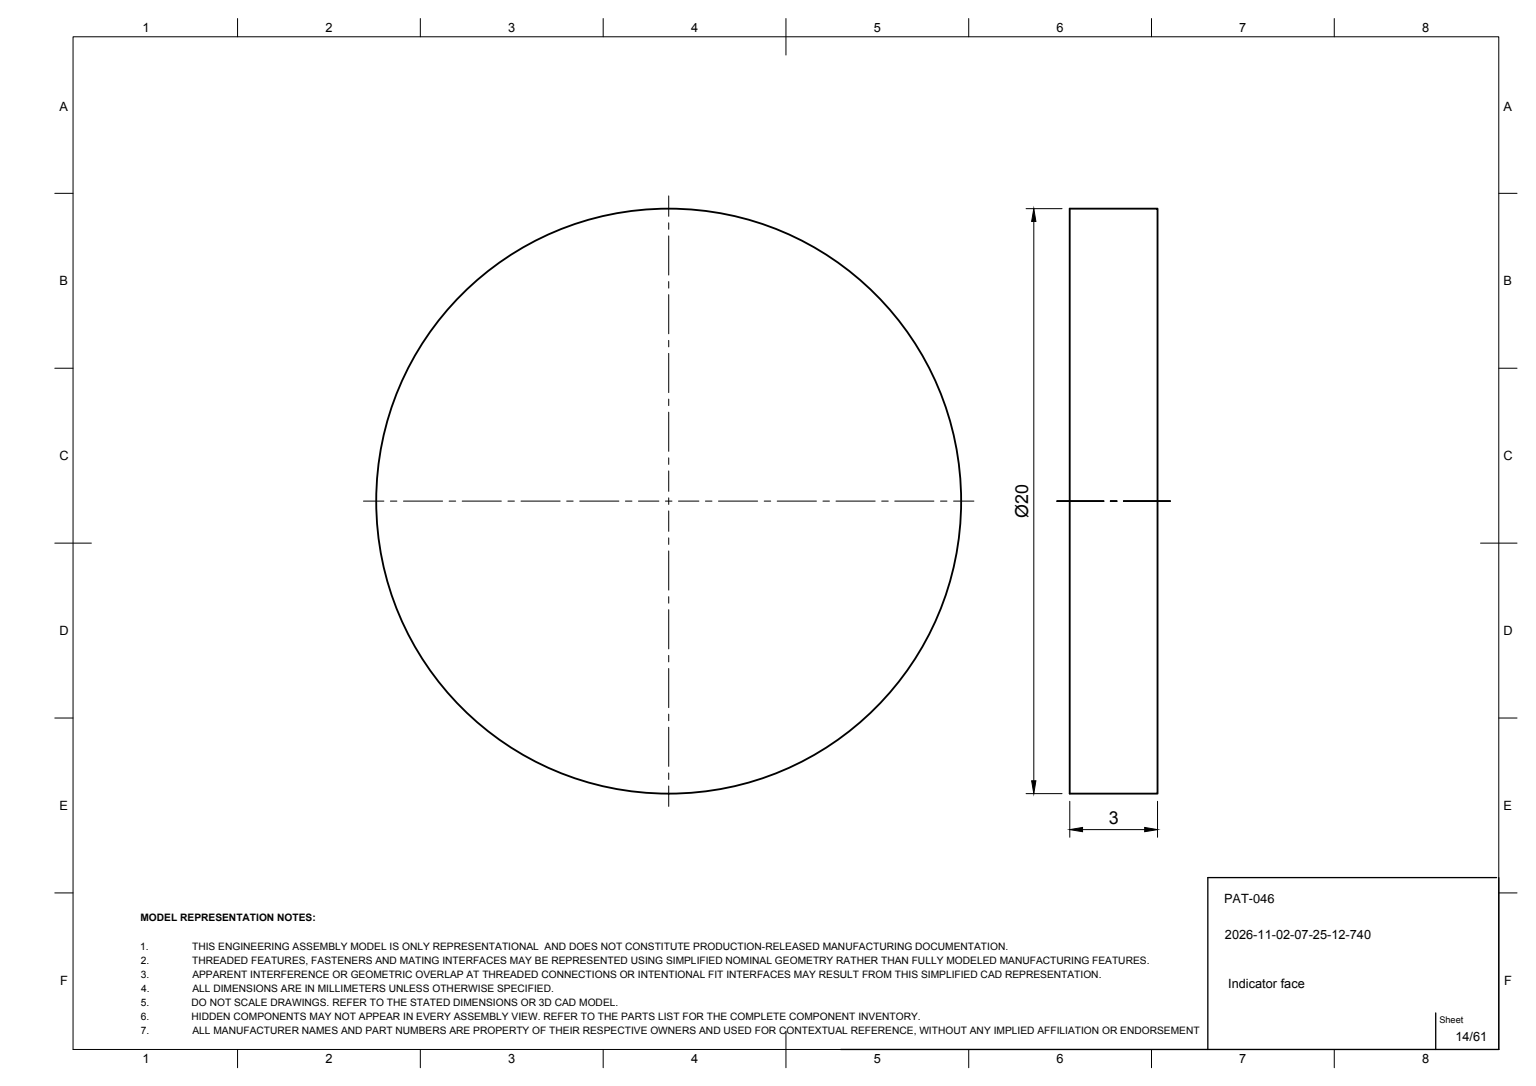
ISO-10303-21;
HEADER;
/* Generated by software containing ST-Developer
 * from STEP Tools, Inc. (www.steptools.com) 
 */

FILE_DESCRIPTION(
/* description */ ('Gear mesh backlash fixture'),
/* implementation_level */ '2;1');

FILE_NAME(
/* name */ 'Indicator face.step',
/* time_stamp */ '2026-10-28T03:26:00-07:00',
/* author */ (''),
/* organization */ (''),
/* preprocessor_version */ 'ST-DEVELOPER v20.2',
/* originating_system */ 'Autodesk Translation Framework v15.17.0.0',
/* authorisation */ '');

FILE_SCHEMA (('AUTOMOTIVE_DESIGN { 1 0 10303 214 3 1 1 }'));
ENDSEC;

DATA;
#10=MECHANICAL_DESIGN_GEOMETRIC_PRESENTATION_REPRESENTATION('',(#1025),#57900);
#925=SHAPE_REPRESENTATION_RELATIONSHIP('SRR','None',#58120,#975);
#975=ADVANCED_BREP_SHAPE_REPRESENTATION('',(#1090),#57853);
#1025=STYLED_ITEM('',(#58458),#1090);
#1090=MANIFOLD_SOLID_BREP('Body1',#13585);
#1391=PLANE('',#14445);
#1392=PLANE('',#14446);
#1808=FACE_OUTER_BOUND('',#2635,.T.);
#1809=FACE_OUTER_BOUND('',#2636,.T.);
#1810=FACE_OUTER_BOUND('',#2637,.T.);
#2635=EDGE_LOOP('',(#9415,#9416,#9417,#9418));
#2636=EDGE_LOOP('',(#9419));
#2637=EDGE_LOOP('',(#9420));
#3551=LINE('',#19900,#4440);
#4440=VECTOR('',#16216,1.);
#5310=CIRCLE('',#14443,1.);
#5311=CIRCLE('',#14444,1.);
#5955=VERTEX_POINT('',#19897);
#5956=VERTEX_POINT('',#19899);
#7294=EDGE_CURVE('',#5955,#5955,#5310,.T.);
#7295=EDGE_CURVE('',#5955,#5956,#3551,.T.);
#7296=EDGE_CURVE('',#5956,#5956,#5311,.T.);
#9415=ORIENTED_EDGE('',*,*,#7294,.F.);
#9416=ORIENTED_EDGE('',*,*,#7295,.T.);
#9417=ORIENTED_EDGE('',*,*,#7296,.T.);
#9418=ORIENTED_EDGE('',*,*,#7295,.F.);
#9419=ORIENTED_EDGE('',*,*,#7294,.T.);
#9420=ORIENTED_EDGE('',*,*,#7296,.F.);
#12638=CYLINDRICAL_SURFACE('',#14442,1.);
#12925=ADVANCED_FACE('',(#1808),#12638,.T.);
#12926=ADVANCED_FACE('',(#1809),#1391,.T.);
#12927=ADVANCED_FACE('',(#1810),#1392,.F.);
#13585=CLOSED_SHELL('',(#12925,#12926,#12927));
#14441=AXIS2_PLACEMENT_3D('',#19895,#16210,#16211);
#14442=AXIS2_PLACEMENT_3D('',#19896,#16212,#16213);
#14443=AXIS2_PLACEMENT_3D('',#19898,#16214,#16215);
#14444=AXIS2_PLACEMENT_3D('',#19901,#16217,#16218);
#14445=AXIS2_PLACEMENT_3D('',#19902,#16219,#16220);
#14446=AXIS2_PLACEMENT_3D('',#19903,#16221,#16222);
#16210=DIRECTION('axis',(0.,0.,1.));
#16211=DIRECTION('refdir',(1.,0.,0.));
#16212=DIRECTION('center_axis',(0.,1.,0.));
#16213=DIRECTION('ref_axis',(1.,0.,0.));
#16214=DIRECTION('center_axis',(0.,1.,0.));
#16215=DIRECTION('ref_axis',(1.,0.,0.));
#16216=DIRECTION('',(0.,-1.,0.));
#16217=DIRECTION('center_axis',(0.,1.,0.));
#16218=DIRECTION('ref_axis',(1.,0.,0.));
#16219=DIRECTION('center_axis',(0.,1.,0.));
#16220=DIRECTION('ref_axis',(1.,0.,0.));
#16221=DIRECTION('center_axis',(0.,1.,0.));
#16222=DIRECTION('ref_axis',(1.,0.,0.));
#19895=CARTESIAN_POINT('',(0.,0.,0.));
#19896=CARTESIAN_POINT('Origin',(6.,10.,12.));
#19897=CARTESIAN_POINT('',(5.,10.3,12.));
#19898=CARTESIAN_POINT('Origin',(6.,10.3,12.));
#19899=CARTESIAN_POINT('',(5.,10.,12.));
#19900=CARTESIAN_POINT('',(5.,10.,12.));
#19901=CARTESIAN_POINT('Origin',(6.,10.,12.));
#19902=CARTESIAN_POINT('Origin',(6.,10.3,12.));
#19903=CARTESIAN_POINT('Origin',(6.,10.,12.));
#57794=UNCERTAINTY_MEASURE_WITH_UNIT(LENGTH_MEASURE(0.001),#57901,
'DISTANCE_ACCURACY_VALUE',
'Maximum model space distance between geometric entities at asserted c
onnectivities');
#57841=UNCERTAINTY_MEASURE_WITH_UNIT(LENGTH_MEASURE(0.001),#57901,
'DISTANCE_ACCURACY_VALUE',
'Maximum model space distance between geometric entities at asserted c
onnectivities');
#57853=(
GEOMETRIC_REPRESENTATION_CONTEXT(3)
GLOBAL_UNCERTAINTY_ASSIGNED_CONTEXT((#57794))
GLOBAL_UNIT_ASSIGNED_CONTEXT((#57901,#57903,#57904))
REPRESENTATION_CONTEXT('','3D')
);
#57900=(
GEOMETRIC_REPRESENTATION_CONTEXT(3)
GLOBAL_UNCERTAINTY_ASSIGNED_CONTEXT((#57841))
GLOBAL_UNIT_ASSIGNED_CONTEXT((#57901,#57903,#57904))
REPRESENTATION_CONTEXT('','3D')
);
#57901=(
LENGTH_UNIT()
NAMED_UNIT(*)
SI_UNIT(.CENTI.,.METRE.)
);
#57903=(
NAMED_UNIT(*)
PLANE_ANGLE_UNIT()
SI_UNIT($,.RADIAN.)
);
#57904=(
NAMED_UNIT(*)
SI_UNIT($,.STERADIAN.)
SOLID_ANGLE_UNIT()
);
#57916=SHAPE_DEFINITION_REPRESENTATION(#57974,#58120);
#57974=PRODUCT_DEFINITION_SHAPE('',$,#58179);
#58120=SHAPE_REPRESENTATION('',(#14441),#57853);
#58167=PRODUCT_DEFINITION_CONTEXT('part definition',#58343,'design');
#58179=PRODUCT_DEFINITION('Indicator face','Indicator face',#58237,#58167);
#58237=PRODUCT_DEFINITION_FORMATION('',$,#58356);
#58343=APPLICATION_CONTEXT(
'Core Data for Automotive Mechanical Design Process');
#58344=PRODUCT_CONTEXT('part definition',#58343,'mechanical');
#58356=PRODUCT('Indicator face','Indicator face','Indicator face',(#58344));
#58452=COLOUR_RGB('Sky Blue',0.24,0.69,0.87);
#58453=FILL_AREA_STYLE_COLOUR('',#58452);
#58454=FILL_AREA_STYLE('',(#58453));
#58455=SURFACE_STYLE_FILL_AREA(#58454);
#58456=SURFACE_SIDE_STYLE('',(#58455));
#58457=SURFACE_STYLE_USAGE(.BOTH.,#58456);
#58458=PRESENTATION_STYLE_ASSIGNMENT((#58457));
ENDSEC;
END-ISO-10303-21;
